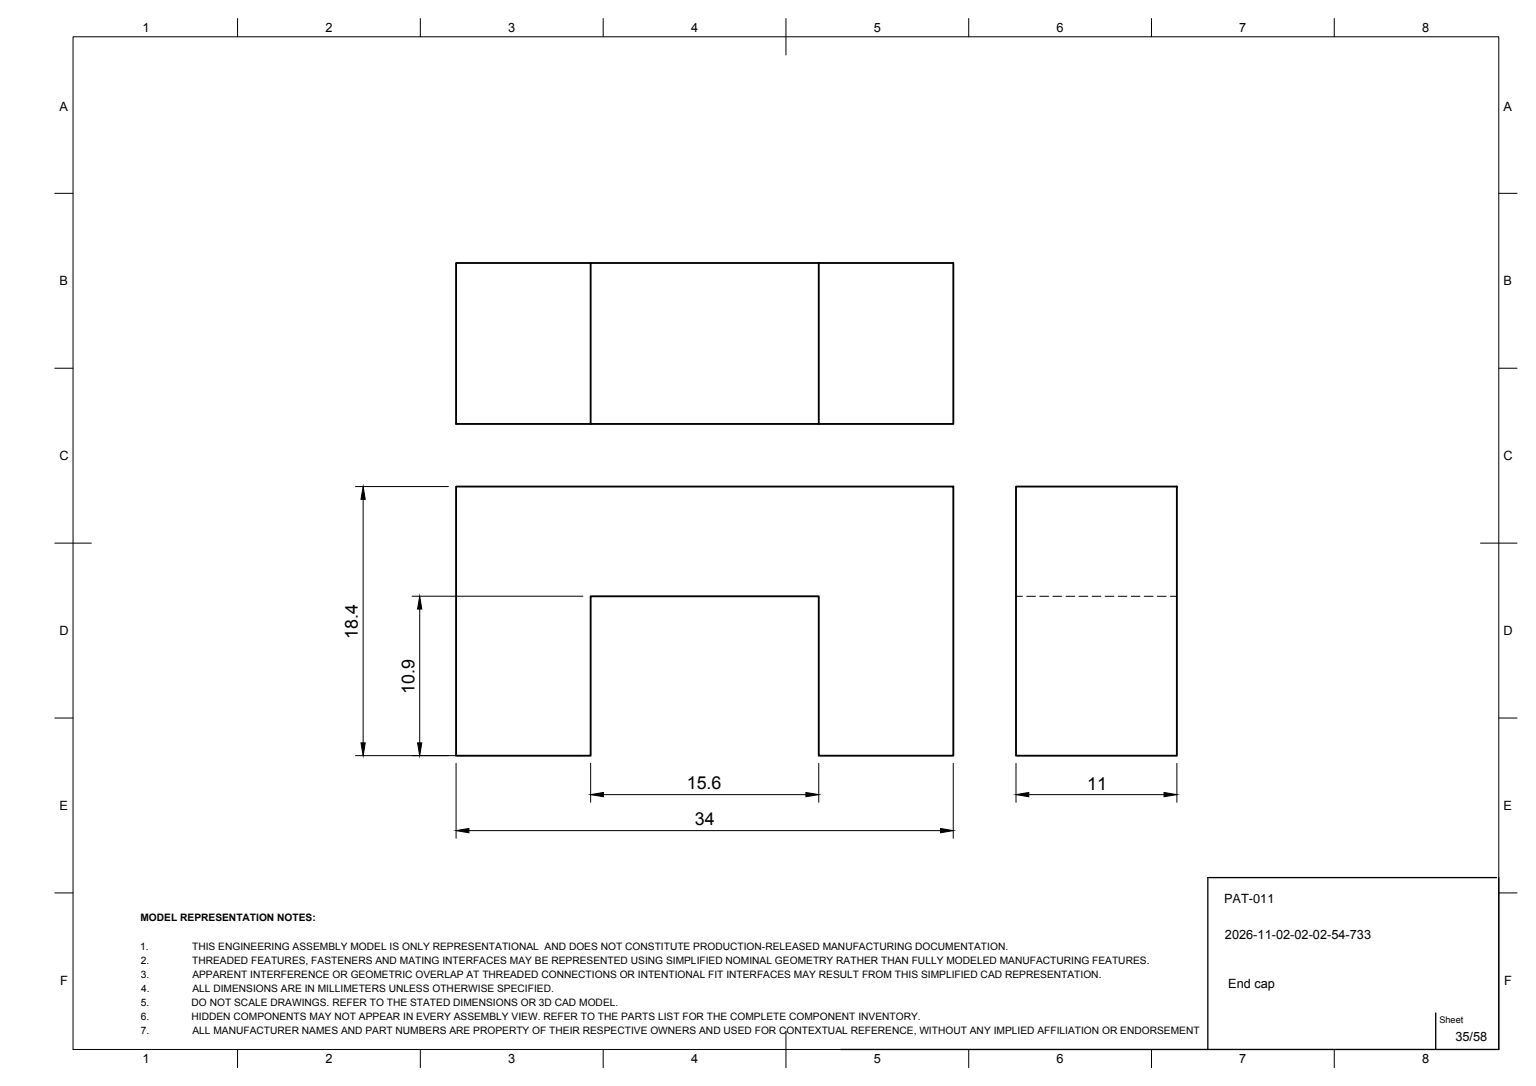
ISO-10303-21;
HEADER;
/* Generated by software containing ST-Developer
 * from STEP Tools, Inc. (www.steptools.com) 
 */

FILE_DESCRIPTION(
/* description */ ('Belt tension measurement rig'),
/* implementation_level */ '2;1');

FILE_NAME(
/* name */ 'End cap.step',
/* time_stamp */ '2026-10-28T03:24:44-07:00',
/* author */ (''),
/* organization */ (''),
/* preprocessor_version */ 'ST-DEVELOPER v20.2',
/* originating_system */ 'Autodesk Translation Framework v15.17.0.0',
/* authorisation */ '');

FILE_SCHEMA (('AUTOMOTIVE_DESIGN { 1 0 10303 214 3 1 1 }'));
ENDSEC;

DATA;
#10=MECHANICAL_DESIGN_GEOMETRIC_PRESENTATION_REPRESENTATION('',(#729),#23587);
#611=SHAPE_REPRESENTATION_RELATIONSHIP('SRR','None',#23859,#666);
#666=ADVANCED_BREP_SHAPE_REPRESENTATION('',(#799),#23557);
#729=STYLED_ITEM('',(#24225),#799);
#799=MANIFOLD_SOLID_BREP('Body1',#12234);
#1229=PLANE('',#13616);
#1230=PLANE('',#13617);
#1231=PLANE('',#13618);
#1232=PLANE('',#13619);
#1233=PLANE('',#13620);
#1234=PLANE('',#13621);
#1235=PLANE('',#13622);
#1236=PLANE('',#13623);
#1237=PLANE('',#13624);
#1238=PLANE('',#13625);
#1709=FACE_OUTER_BOUND('',#2557,.T.);
#1710=FACE_OUTER_BOUND('',#2558,.T.);
#1711=FACE_OUTER_BOUND('',#2559,.T.);
#1712=FACE_OUTER_BOUND('',#2560,.T.);
#1713=FACE_OUTER_BOUND('',#2561,.T.);
#1714=FACE_OUTER_BOUND('',#2562,.T.);
#1715=FACE_OUTER_BOUND('',#2563,.T.);
#1716=FACE_OUTER_BOUND('',#2564,.T.);
#1717=FACE_OUTER_BOUND('',#2565,.T.);
#1718=FACE_OUTER_BOUND('',#2566,.T.);
#2557=EDGE_LOOP('',(#9554,#9555,#9556,#9557));
#2558=EDGE_LOOP('',(#9558,#9559,#9560,#9561));
#2559=EDGE_LOOP('',(#9562,#9563,#9564,#9565));
#2560=EDGE_LOOP('',(#9566,#9567,#9568,#9569));
#2561=EDGE_LOOP('',(#9570,#9571,#9572,#9573));
#2562=EDGE_LOOP('',(#9574,#9575,#9576,#9577));
#2563=EDGE_LOOP('',(#9578,#9579,#9580,#9581));
#2564=EDGE_LOOP('',(#9582,#9583,#9584,#9585));
#2565=EDGE_LOOP('',(#9586,#9587,#9588,#9589,#9590,#9591,#9592,#9593));
#2566=EDGE_LOOP('',(#9594,#9595,#9596,#9597,#9598,#9599,#9600,#9601));
#3407=LINE('',#20733,#4158);
#3408=LINE('',#20735,#4159);
#3409=LINE('',#20737,#4160);
#3410=LINE('',#20738,#4161);
#3411=LINE('',#20741,#4162);
#3412=LINE('',#20743,#4163);
#3413=LINE('',#20744,#4164);
#3414=LINE('',#20747,#4165);
#3415=LINE('',#20749,#4166);
#3416=LINE('',#20750,#4167);
#3417=LINE('',#20753,#4168);
#3418=LINE('',#20755,#4169);
#3419=LINE('',#20756,#4170);
#3420=LINE('',#20759,#4171);
#3421=LINE('',#20761,#4172);
#3422=LINE('',#20762,#4173);
#3423=LINE('',#20765,#4174);
#3424=LINE('',#20767,#4175);
#3425=LINE('',#20768,#4176);
#3426=LINE('',#20771,#4177);
#3427=LINE('',#20773,#4178);
#3428=LINE('',#20774,#4179);
#3429=LINE('',#20776,#4180);
#3430=LINE('',#20777,#4181);
#4158=VECTOR('',#16438,1.);
#4159=VECTOR('',#16439,1.);
#4160=VECTOR('',#16440,1.);
#4161=VECTOR('',#16441,1.);
#4162=VECTOR('',#16444,1.);
#4163=VECTOR('',#16445,1.);
#4164=VECTOR('',#16446,1.);
#4165=VECTOR('',#16449,1.);
#4166=VECTOR('',#16450,1.);
#4167=VECTOR('',#16451,1.);
#4168=VECTOR('',#16454,1.);
#4169=VECTOR('',#16455,1.);
#4170=VECTOR('',#16456,1.);
#4171=VECTOR('',#16459,1.);
#4172=VECTOR('',#16460,1.);
#4173=VECTOR('',#16461,1.);
#4174=VECTOR('',#16464,1.);
#4175=VECTOR('',#16465,1.);
#4176=VECTOR('',#16466,1.);
#4177=VECTOR('',#16469,1.);
#4178=VECTOR('',#16470,1.);
#4179=VECTOR('',#16471,1.);
#4180=VECTOR('',#16474,1.);
#4181=VECTOR('',#16475,1.);
#5783=VERTEX_POINT('',#20731);
#5784=VERTEX_POINT('',#20732);
#5785=VERTEX_POINT('',#20734);
#5786=VERTEX_POINT('',#20736);
#5787=VERTEX_POINT('',#20740);
#5788=VERTEX_POINT('',#20742);
#5789=VERTEX_POINT('',#20746);
#5790=VERTEX_POINT('',#20748);
#5791=VERTEX_POINT('',#20752);
#5792=VERTEX_POINT('',#20754);
#5793=VERTEX_POINT('',#20758);
#5794=VERTEX_POINT('',#20760);
#5795=VERTEX_POINT('',#20764);
#5796=VERTEX_POINT('',#20766);
#5797=VERTEX_POINT('',#20770);
#5798=VERTEX_POINT('',#20772);
#7136=EDGE_CURVE('',#5783,#5784,#3407,.T.);
#7137=EDGE_CURVE('',#5783,#5785,#3408,.T.);
#7138=EDGE_CURVE('',#5786,#5785,#3409,.T.);
#7139=EDGE_CURVE('',#5784,#5786,#3410,.T.);
#7140=EDGE_CURVE('',#5784,#5787,#3411,.T.);
#7141=EDGE_CURVE('',#5788,#5786,#3412,.T.);
#7142=EDGE_CURVE('',#5787,#5788,#3413,.T.);
#7143=EDGE_CURVE('',#5787,#5789,#3414,.T.);
#7144=EDGE_CURVE('',#5790,#5788,#3415,.T.);
#7145=EDGE_CURVE('',#5789,#5790,#3416,.T.);
#7146=EDGE_CURVE('',#5789,#5791,#3417,.T.);
#7147=EDGE_CURVE('',#5792,#5790,#3418,.T.);
#7148=EDGE_CURVE('',#5791,#5792,#3419,.T.);
#7149=EDGE_CURVE('',#5791,#5793,#3420,.T.);
#7150=EDGE_CURVE('',#5794,#5792,#3421,.T.);
#7151=EDGE_CURVE('',#5793,#5794,#3422,.T.);
#7152=EDGE_CURVE('',#5793,#5795,#3423,.T.);
#7153=EDGE_CURVE('',#5796,#5794,#3424,.T.);
#7154=EDGE_CURVE('',#5795,#5796,#3425,.T.);
#7155=EDGE_CURVE('',#5795,#5797,#3426,.T.);
#7156=EDGE_CURVE('',#5798,#5796,#3427,.T.);
#7157=EDGE_CURVE('',#5797,#5798,#3428,.T.);
#7158=EDGE_CURVE('',#5797,#5783,#3429,.T.);
#7159=EDGE_CURVE('',#5785,#5798,#3430,.T.);
#9554=ORIENTED_EDGE('',*,*,#7136,.F.);
#9555=ORIENTED_EDGE('',*,*,#7137,.T.);
#9556=ORIENTED_EDGE('',*,*,#7138,.F.);
#9557=ORIENTED_EDGE('',*,*,#7139,.F.);
#9558=ORIENTED_EDGE('',*,*,#7140,.F.);
#9559=ORIENTED_EDGE('',*,*,#7139,.T.);
#9560=ORIENTED_EDGE('',*,*,#7141,.F.);
#9561=ORIENTED_EDGE('',*,*,#7142,.F.);
#9562=ORIENTED_EDGE('',*,*,#7143,.F.);
#9563=ORIENTED_EDGE('',*,*,#7142,.T.);
#9564=ORIENTED_EDGE('',*,*,#7144,.F.);
#9565=ORIENTED_EDGE('',*,*,#7145,.F.);
#9566=ORIENTED_EDGE('',*,*,#7146,.F.);
#9567=ORIENTED_EDGE('',*,*,#7145,.T.);
#9568=ORIENTED_EDGE('',*,*,#7147,.F.);
#9569=ORIENTED_EDGE('',*,*,#7148,.F.);
#9570=ORIENTED_EDGE('',*,*,#7149,.F.);
#9571=ORIENTED_EDGE('',*,*,#7148,.T.);
#9572=ORIENTED_EDGE('',*,*,#7150,.F.);
#9573=ORIENTED_EDGE('',*,*,#7151,.F.);
#9574=ORIENTED_EDGE('',*,*,#7152,.F.);
#9575=ORIENTED_EDGE('',*,*,#7151,.T.);
#9576=ORIENTED_EDGE('',*,*,#7153,.F.);
#9577=ORIENTED_EDGE('',*,*,#7154,.F.);
#9578=ORIENTED_EDGE('',*,*,#7155,.F.);
#9579=ORIENTED_EDGE('',*,*,#7154,.T.);
#9580=ORIENTED_EDGE('',*,*,#7156,.F.);
#9581=ORIENTED_EDGE('',*,*,#7157,.F.);
#9582=ORIENTED_EDGE('',*,*,#7158,.F.);
#9583=ORIENTED_EDGE('',*,*,#7157,.T.);
#9584=ORIENTED_EDGE('',*,*,#7159,.F.);
#9585=ORIENTED_EDGE('',*,*,#7137,.F.);
#9586=ORIENTED_EDGE('',*,*,#7158,.T.);
#9587=ORIENTED_EDGE('',*,*,#7136,.T.);
#9588=ORIENTED_EDGE('',*,*,#7140,.T.);
#9589=ORIENTED_EDGE('',*,*,#7143,.T.);
#9590=ORIENTED_EDGE('',*,*,#7146,.T.);
#9591=ORIENTED_EDGE('',*,*,#7149,.T.);
#9592=ORIENTED_EDGE('',*,*,#7152,.T.);
#9593=ORIENTED_EDGE('',*,*,#7155,.T.);
#9594=ORIENTED_EDGE('',*,*,#7159,.T.);
#9595=ORIENTED_EDGE('',*,*,#7156,.T.);
#9596=ORIENTED_EDGE('',*,*,#7153,.T.);
#9597=ORIENTED_EDGE('',*,*,#7150,.T.);
#9598=ORIENTED_EDGE('',*,*,#7147,.T.);
#9599=ORIENTED_EDGE('',*,*,#7144,.T.);
#9600=ORIENTED_EDGE('',*,*,#7141,.T.);
#9601=ORIENTED_EDGE('',*,*,#7138,.T.);
#11850=ADVANCED_FACE('',(#1709),#1229,.T.);
#11851=ADVANCED_FACE('',(#1710),#1230,.T.);
#11852=ADVANCED_FACE('',(#1711),#1231,.T.);
#11853=ADVANCED_FACE('',(#1712),#1232,.T.);
#11854=ADVANCED_FACE('',(#1713),#1233,.T.);
#11855=ADVANCED_FACE('',(#1714),#1234,.T.);
#11856=ADVANCED_FACE('',(#1715),#1235,.T.);
#11857=ADVANCED_FACE('',(#1716),#1236,.T.);
#11858=ADVANCED_FACE('',(#1717),#1237,.T.);
#11859=ADVANCED_FACE('',(#1718),#1238,.T.);
#12234=CLOSED_SHELL('',(#11850,#11851,#11852,#11853,#11854,#11855,#11856,
#11857,#11858,#11859));
#13615=AXIS2_PLACEMENT_3D('',#20729,#16434,#16435);
#13616=AXIS2_PLACEMENT_3D('',#20730,#16436,#16437);
#13617=AXIS2_PLACEMENT_3D('',#20739,#16442,#16443);
#13618=AXIS2_PLACEMENT_3D('',#20745,#16447,#16448);
#13619=AXIS2_PLACEMENT_3D('',#20751,#16452,#16453);
#13620=AXIS2_PLACEMENT_3D('',#20757,#16457,#16458);
#13621=AXIS2_PLACEMENT_3D('',#20763,#16462,#16463);
#13622=AXIS2_PLACEMENT_3D('',#20769,#16467,#16468);
#13623=AXIS2_PLACEMENT_3D('',#20775,#16472,#16473);
#13624=AXIS2_PLACEMENT_3D('',#20778,#16476,#16477);
#13625=AXIS2_PLACEMENT_3D('',#20779,#16478,#16479);
#16434=DIRECTION('axis',(0.,0.,1.));
#16435=DIRECTION('refdir',(1.,0.,0.));
#16436=DIRECTION('center_axis',(0.,0.,-1.));
#16437=DIRECTION('ref_axis',(0.,-1.,0.));
#16438=DIRECTION('',(0.,1.,0.));
#16439=DIRECTION('',(-1.,0.,0.));
#16440=DIRECTION('',(0.,-1.,0.));
#16441=DIRECTION('',(-1.,0.,0.));
#16442=DIRECTION('center_axis',(0.,1.,0.));
#16443=DIRECTION('ref_axis',(0.,0.,-1.));
#16444=DIRECTION('',(0.,0.,1.));
#16445=DIRECTION('',(0.,0.,-1.));
#16446=DIRECTION('',(-1.,0.,0.));
#16447=DIRECTION('center_axis',(0.,0.,-1.));
#16448=DIRECTION('ref_axis',(0.,-1.,0.));
#16449=DIRECTION('',(0.,1.,0.));
#16450=DIRECTION('',(0.,-1.,0.));
#16451=DIRECTION('',(-1.,0.,0.));
#16452=DIRECTION('center_axis',(0.,-1.,0.));
#16453=DIRECTION('ref_axis',(0.,0.,1.));
#16454=DIRECTION('',(0.,0.,-1.));
#16455=DIRECTION('',(0.,0.,1.));
#16456=DIRECTION('',(-1.,0.,0.));
#16457=DIRECTION('center_axis',(0.,0.,-1.));
#16458=DIRECTION('ref_axis',(0.,-1.,0.));
#16459=DIRECTION('',(0.,1.,0.));
#16460=DIRECTION('',(0.,-1.,0.));
#16461=DIRECTION('',(-1.,0.,0.));
#16462=DIRECTION('center_axis',(0.,1.,0.));
#16463=DIRECTION('ref_axis',(0.,0.,-1.));
#16464=DIRECTION('',(0.,0.,1.));
#16465=DIRECTION('',(0.,0.,-1.));
#16466=DIRECTION('',(-1.,0.,0.));
#16467=DIRECTION('center_axis',(0.,0.,1.));
#16468=DIRECTION('ref_axis',(0.,1.,0.));
#16469=DIRECTION('',(0.,-1.,0.));
#16470=DIRECTION('',(0.,1.,0.));
#16471=DIRECTION('',(-1.,0.,0.));
#16472=DIRECTION('center_axis',(0.,-1.,0.));
#16473=DIRECTION('ref_axis',(0.,0.,1.));
#16474=DIRECTION('',(0.,0.,-1.));
#16475=DIRECTION('',(0.,0.,1.));
#16476=DIRECTION('center_axis',(1.,0.,0.));
#16477=DIRECTION('ref_axis',(0.,0.,-1.));
#16478=DIRECTION('center_axis',(-1.,0.,0.));
#16479=DIRECTION('ref_axis',(0.,0.,1.));
#20729=CARTESIAN_POINT('',(0.,0.,0.));
#20730=CARTESIAN_POINT('Origin',(-1.97,-0.78,0.46));
#20731=CARTESIAN_POINT('',(-1.97,-1.7,0.46));
#20732=CARTESIAN_POINT('',(-1.97,-0.78,0.46));
#20733=CARTESIAN_POINT('',(-1.97,-1.7,0.46));
#20734=CARTESIAN_POINT('',(-3.07,-1.7,0.46));
#20735=CARTESIAN_POINT('',(-1.97,-1.7,0.46));
#20736=CARTESIAN_POINT('',(-3.07,-0.78,0.46));
#20737=CARTESIAN_POINT('',(-3.07,-1.7,0.46));
#20738=CARTESIAN_POINT('',(-1.97,-0.78,0.46));
#20739=CARTESIAN_POINT('Origin',(-1.97,-0.78,1.55));
#20740=CARTESIAN_POINT('',(-1.97,-0.78,1.55));
#20741=CARTESIAN_POINT('',(-1.97,-0.78,0.46));
#20742=CARTESIAN_POINT('',(-3.07,-0.78,1.55));
#20743=CARTESIAN_POINT('',(-3.07,-0.78,0.46));
#20744=CARTESIAN_POINT('',(-1.97,-0.78,1.55));
#20745=CARTESIAN_POINT('Origin',(-1.97,0.78,1.55));
#20746=CARTESIAN_POINT('',(-1.97,0.78,1.55));
#20747=CARTESIAN_POINT('',(-1.97,-0.78,1.55));
#20748=CARTESIAN_POINT('',(-3.07,0.78,1.55));
#20749=CARTESIAN_POINT('',(-3.07,-0.78,1.55));
#20750=CARTESIAN_POINT('',(-1.97,0.78,1.55));
#20751=CARTESIAN_POINT('Origin',(-1.97,0.78,0.46));
#20752=CARTESIAN_POINT('',(-1.97,0.78,0.46));
#20753=CARTESIAN_POINT('',(-1.97,0.78,1.55));
#20754=CARTESIAN_POINT('',(-3.07,0.78,0.46));
#20755=CARTESIAN_POINT('',(-3.07,0.78,1.55));
#20756=CARTESIAN_POINT('',(-1.97,0.78,0.46));
#20757=CARTESIAN_POINT('Origin',(-1.97,1.7,0.46));
#20758=CARTESIAN_POINT('',(-1.97,1.7,0.46));
#20759=CARTESIAN_POINT('',(-1.97,0.78,0.46));
#20760=CARTESIAN_POINT('',(-3.07,1.7,0.46));
#20761=CARTESIAN_POINT('',(-3.07,0.78,0.46));
#20762=CARTESIAN_POINT('',(-1.97,1.7,0.46));
#20763=CARTESIAN_POINT('Origin',(-1.97,1.7,2.3));
#20764=CARTESIAN_POINT('',(-1.97,1.7,2.3));
#20765=CARTESIAN_POINT('',(-1.97,1.7,0.46));
#20766=CARTESIAN_POINT('',(-3.07,1.7,2.3));
#20767=CARTESIAN_POINT('',(-3.07,1.7,0.46));
#20768=CARTESIAN_POINT('',(-1.97,1.7,2.3));
#20769=CARTESIAN_POINT('Origin',(-1.97,-1.7,2.3));
#20770=CARTESIAN_POINT('',(-1.97,-1.7,2.3));
#20771=CARTESIAN_POINT('',(-1.97,1.7,2.3));
#20772=CARTESIAN_POINT('',(-3.07,-1.7,2.3));
#20773=CARTESIAN_POINT('',(-3.07,1.7,2.3));
#20774=CARTESIAN_POINT('',(-1.97,-1.7,2.3));
#20775=CARTESIAN_POINT('Origin',(-1.97,-1.7,0.46));
#20776=CARTESIAN_POINT('',(-1.97,-1.7,2.3));
#20777=CARTESIAN_POINT('',(-3.07,-1.7,2.3));
#20778=CARTESIAN_POINT('Origin',(-1.97,0.,1.38));
#20779=CARTESIAN_POINT('Origin',(-3.07,0.,1.38));
#23492=UNCERTAINTY_MEASURE_WITH_UNIT(LENGTH_MEASURE(0.001),#23588,
'DISTANCE_ACCURACY_VALUE',
'Maximum model space distance between geometric entities at asserted c
onnectivities');
#23522=UNCERTAINTY_MEASURE_WITH_UNIT(LENGTH_MEASURE(0.001),#23588,
'DISTANCE_ACCURACY_VALUE',
'Maximum model space distance between geometric entities at asserted c
onnectivities');
#23557=(
GEOMETRIC_REPRESENTATION_CONTEXT(3)
GLOBAL_UNCERTAINTY_ASSIGNED_CONTEXT((#23492))
GLOBAL_UNIT_ASSIGNED_CONTEXT((#23588,#23590,#23591))
REPRESENTATION_CONTEXT('','3D')
);
#23587=(
GEOMETRIC_REPRESENTATION_CONTEXT(3)
GLOBAL_UNCERTAINTY_ASSIGNED_CONTEXT((#23522))
GLOBAL_UNIT_ASSIGNED_CONTEXT((#23588,#23590,#23591))
REPRESENTATION_CONTEXT('','3D')
);
#23588=(
LENGTH_UNIT()
NAMED_UNIT(*)
SI_UNIT(.CENTI.,.METRE.)
);
#23590=(
NAMED_UNIT(*)
PLANE_ANGLE_UNIT()
SI_UNIT($,.RADIAN.)
);
#23591=(
NAMED_UNIT(*)
SI_UNIT($,.STERADIAN.)
SOLID_ANGLE_UNIT()
);
#23626=SHAPE_DEFINITION_REPRESENTATION(#23695,#23859);
#23695=PRODUCT_DEFINITION_SHAPE('',$,#23924);
#23859=SHAPE_REPRESENTATION('',(#13615),#23557);
#23889=PRODUCT_DEFINITION_CONTEXT('part definition',#24083,'design');
#23924=PRODUCT_DEFINITION('End cap','End cap',#23988,#23889);
#23988=PRODUCT_DEFINITION_FORMATION('',$,#24119);
#24083=APPLICATION_CONTEXT(
'Core Data for Automotive Mechanical Design Process');
#24084=PRODUCT_CONTEXT('part definition',#24083,'mechanical');
#24119=PRODUCT('End cap','End cap','End cap',(#24084));
#24219=COLOUR_RGB('Off White',0.89,0.88,0.83);
#24220=FILL_AREA_STYLE_COLOUR('',#24219);
#24221=FILL_AREA_STYLE('',(#24220));
#24222=SURFACE_STYLE_FILL_AREA(#24221);
#24223=SURFACE_SIDE_STYLE('',(#24222));
#24224=SURFACE_STYLE_USAGE(.BOTH.,#24223);
#24225=PRESENTATION_STYLE_ASSIGNMENT((#24224));
ENDSEC;
END-ISO-10303-21;
